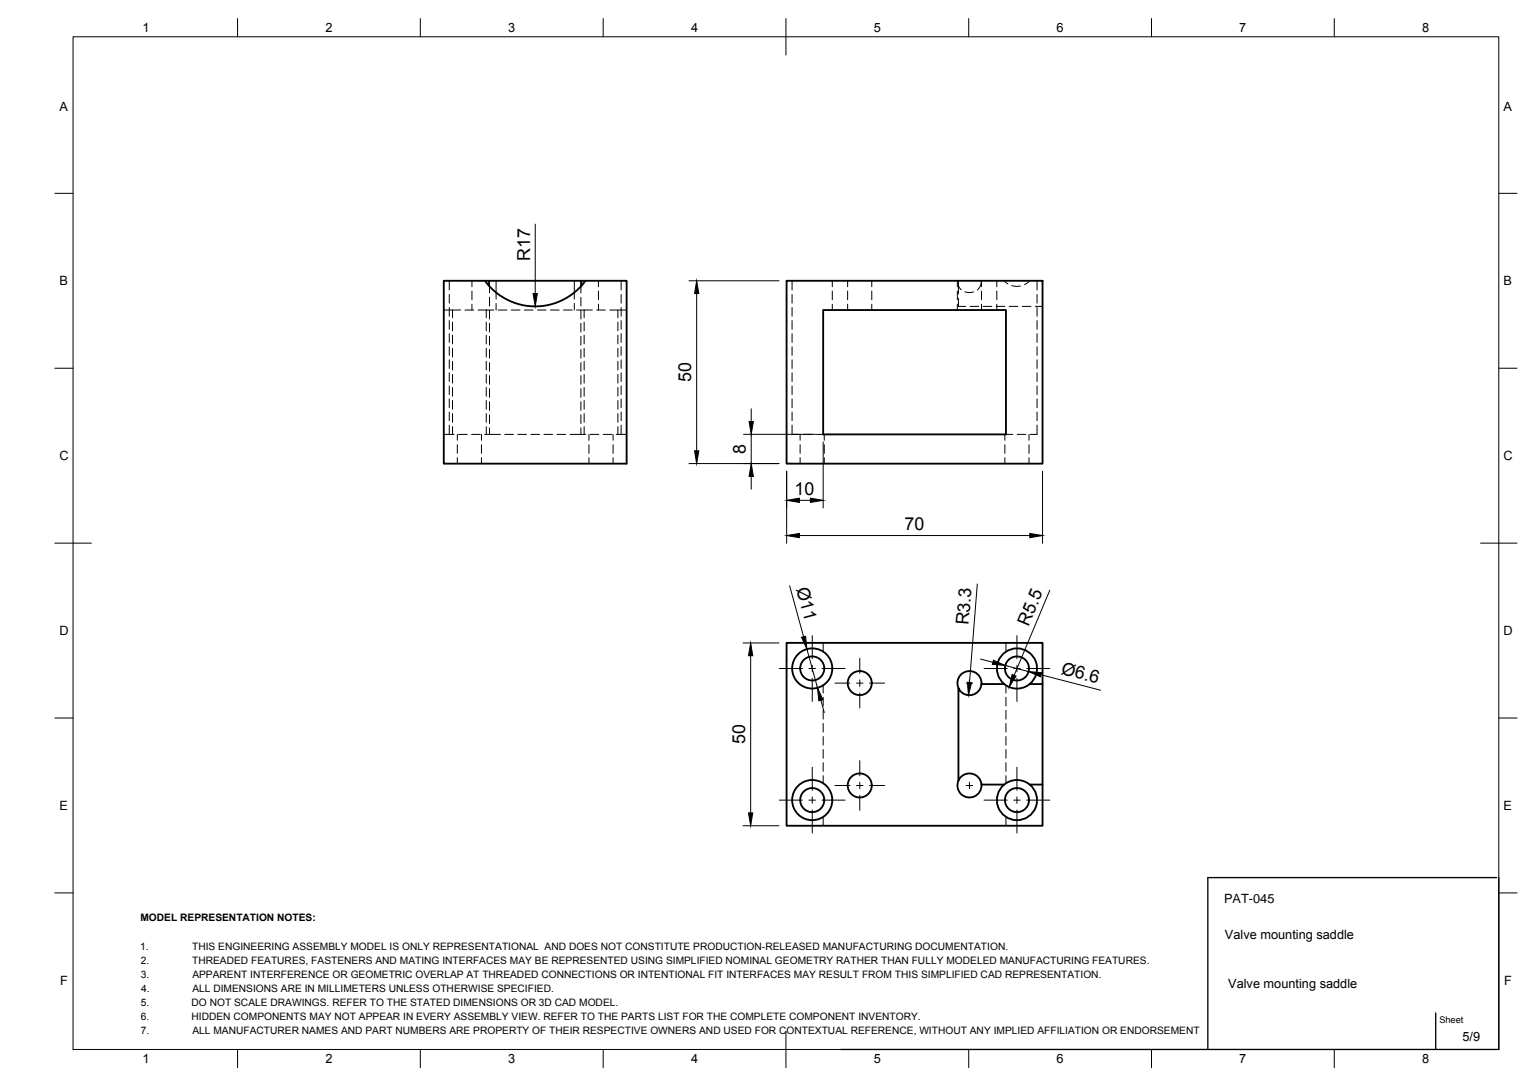
ISO-10303-21;
HEADER;
/* Generated by software containing ST-Developer
 * from STEP Tools, Inc. (www.steptools.com) 
 */

FILE_DESCRIPTION(
/* description */ ('Gauge isolation and snubber set'),
/* implementation_level */ '2;1');

FILE_NAME(
/* name */ 'Valve mounting saddle.step',
/* time_stamp */ '2026-10-29T16:58:15-07:00',
/* author */ (''),
/* organization */ (''),
/* preprocessor_version */ 'ST-DEVELOPER v20.2',
/* originating_system */ 'Autodesk Translation Framework v15.17.0.0',
/* authorisation */ '');

FILE_SCHEMA (('AUTOMOTIVE_DESIGN { 1 0 10303 214 3 1 1 }'));
ENDSEC;

DATA;
#10=MECHANICAL_DESIGN_GEOMETRIC_PRESENTATION_REPRESENTATION('',(#94),#4043);
#78=SHAPE_REPRESENTATION_RELATIONSHIP('SRR','None',#4085,#86);
#86=ADVANCED_BREP_SHAPE_REPRESENTATION('',(#104),#4037);
#94=STYLED_ITEM('',(#4211),#104);
#104=MANIFOLD_SOLID_BREP('Body1',#2211);
#128=FACE_BOUND('',#436,.T.);
#129=FACE_BOUND('',#437,.T.);
#130=FACE_BOUND('',#438,.T.);
#131=FACE_BOUND('',#439,.T.);
#132=FACE_BOUND('',#442,.T.);
#133=FACE_BOUND('',#443,.T.);
#134=FACE_BOUND('',#444,.T.);
#135=FACE_BOUND('',#445,.T.);
#136=FACE_BOUND('',#460,.T.);
#137=FACE_BOUND('',#462,.T.);
#138=FACE_BOUND('',#463,.T.);
#139=FACE_BOUND('',#464,.T.);
#140=FACE_BOUND('',#465,.T.);
#141=FACE_BOUND('',#467,.T.);
#142=FACE_BOUND('',#470,.T.);
#143=FACE_BOUND('',#471,.T.);
#144=FACE_BOUND('',#472,.T.);
#145=FACE_BOUND('',#473,.T.);
#160=B_SPLINE_CURVE_WITH_KNOTS('',3,(#3540,#3541,#3542,#3543,#3544,#3545,
#3546,#3547,#3548,#3549,#3550,#3551,#3552,#3553,#3554,#3555,#3556,#3557,
#3558,#3559),.UNSPECIFIED.,.F.,.F.,(4,2,2,2,2,2,2,2,2,4),(2.69569624904958,
2.75192095998156,2.89158432667083,3.02781992201341,3.15222641361202,3.27663290521063,
3.40103939680924,3.52544588840784,3.66168148375042,3.68881758098469),
 .UNSPECIFIED.);
#161=B_SPLINE_CURVE_WITH_KNOTS('',3,(#3563,#3564,#3565,#3566,#3567,#3568,
#3569,#3570,#3571,#3572,#3573,#3574,#3575,#3576),.UNSPECIFIED.,.F.,.F.,
(4,2,2,2,2,2,4),(2.49458037721665,2.67223802177451,2.78657360475194,2.90090918772936,
3.01524477070679,3.12958035368422,3.30723799824207),.UNSPECIFIED.);
#162=B_SPLINE_CURVE_WITH_KNOTS('',3,(#3584,#3585,#3586,#3587,#3588,#3589,
#3590,#3591,#3592,#3593,#3594,#3595,#3596,#3597,#3598),.UNSPECIFIED.,.F.,
 .F.,(4,2,2,3,2,2,4),(-0.40632881051271,-0.228671165954853,-0.114335582977427,
0.,0.114335582977426,0.228671165954853,0.40632881051271),.UNSPECIFIED.);
#163=B_SPLINE_CURVE_WITH_KNOTS('',3,(#3601,#3602,#3603,#3604,#3605,#3606,
#3607,#3608,#3609,#3610,#3611,#3612,#3613,#3614,#3615,#3616,#3617,#3618,
#3619,#3620,#3621),.UNSPECIFIED.,.F.,.F.,(4,2,2,2,3,2,2,2,2,4),(-0.412184675816244,
-0.385048578539797,-0.248812983197217,-0.124406491598609,0.,0.124406491598609,
0.248812983197217,0.385048578539798,0.524711945229068,0.58093665616105),
 .UNSPECIFIED.);
#193=PLANE('',#2401);
#194=PLANE('',#2424);
#195=PLANE('',#2425);
#196=PLANE('',#2435);
#197=PLANE('',#2443);
#198=PLANE('',#2446);
#199=PLANE('',#2447);
#200=PLANE('',#2450);
#201=PLANE('',#2456);
#202=PLANE('',#2461);
#203=PLANE('',#2462);
#204=PLANE('',#2463);
#205=PLANE('',#2464);
#206=PLANE('',#2465);
#207=PLANE('',#2466);
#288=FACE_OUTER_BOUND('',#428,.T.);
#289=FACE_OUTER_BOUND('',#429,.T.);
#290=FACE_OUTER_BOUND('',#430,.T.);
#291=FACE_OUTER_BOUND('',#431,.T.);
#292=FACE_OUTER_BOUND('',#432,.T.);
#293=FACE_OUTER_BOUND('',#433,.T.);
#294=FACE_OUTER_BOUND('',#434,.T.);
#295=FACE_OUTER_BOUND('',#435,.T.);
#296=FACE_OUTER_BOUND('',#440,.T.);
#297=FACE_OUTER_BOUND('',#441,.T.);
#298=FACE_OUTER_BOUND('',#446,.T.);
#299=FACE_OUTER_BOUND('',#447,.T.);
#300=FACE_OUTER_BOUND('',#448,.T.);
#301=FACE_OUTER_BOUND('',#449,.T.);
#302=FACE_OUTER_BOUND('',#450,.T.);
#303=FACE_OUTER_BOUND('',#451,.T.);
#304=FACE_OUTER_BOUND('',#452,.T.);
#305=FACE_OUTER_BOUND('',#453,.T.);
#306=FACE_OUTER_BOUND('',#454,.T.);
#307=FACE_OUTER_BOUND('',#455,.T.);
#308=FACE_OUTER_BOUND('',#456,.T.);
#309=FACE_OUTER_BOUND('',#457,.T.);
#310=FACE_OUTER_BOUND('',#458,.T.);
#311=FACE_OUTER_BOUND('',#459,.T.);
#312=FACE_OUTER_BOUND('',#461,.T.);
#313=FACE_OUTER_BOUND('',#466,.T.);
#314=FACE_OUTER_BOUND('',#468,.T.);
#315=FACE_OUTER_BOUND('',#469,.T.);
#428=EDGE_LOOP('',(#1659,#1660,#1661,#1662));
#429=EDGE_LOOP('',(#1663,#1664,#1665,#1666,#1667,#1668,#1669,#1670,#1671,
#1672));
#430=EDGE_LOOP('',(#1673,#1674,#1675,#1676,#1677,#1678,#1679,#1680,#1681,
#1682));
#431=EDGE_LOOP('',(#1683,#1684,#1685,#1686,#1687,#1688,#1689));
#432=EDGE_LOOP('',(#1690,#1691,#1692,#1693,#1694,#1695,#1696));
#433=EDGE_LOOP('',(#1697,#1698,#1699,#1700,#1701,#1702,#1703,#1704));
#434=EDGE_LOOP('',(#1705,#1706,#1707,#1708));
#435=EDGE_LOOP('',(#1709,#1710,#1711,#1712,#1713,#1714,#1715,#1716,#1717,
#1718,#1719,#1720,#1721,#1722));
#436=EDGE_LOOP('',(#1723));
#437=EDGE_LOOP('',(#1724));
#438=EDGE_LOOP('',(#1725));
#439=EDGE_LOOP('',(#1726));
#440=EDGE_LOOP('',(#1727,#1728,#1729,#1730));
#441=EDGE_LOOP('',(#1731,#1732,#1733,#1734,#1735,#1736,#1737,#1738,#1739,
#1740,#1741,#1742,#1743,#1744));
#442=EDGE_LOOP('',(#1745));
#443=EDGE_LOOP('',(#1746));
#444=EDGE_LOOP('',(#1747));
#445=EDGE_LOOP('',(#1748));
#446=EDGE_LOOP('',(#1749,#1750,#1751,#1752,#1753,#1754,#1755,#1756));
#447=EDGE_LOOP('',(#1757,#1758,#1759,#1760));
#448=EDGE_LOOP('',(#1761,#1762,#1763,#1764));
#449=EDGE_LOOP('',(#1765,#1766,#1767,#1768));
#450=EDGE_LOOP('',(#1769,#1770,#1771,#1772));
#451=EDGE_LOOP('',(#1773,#1774,#1775,#1776));
#452=EDGE_LOOP('',(#1777,#1778,#1779,#1780));
#453=EDGE_LOOP('',(#1781,#1782,#1783,#1784,#1785,#1786,#1787,#1788,#1789,
#1790));
#454=EDGE_LOOP('',(#1791,#1792,#1793,#1794));
#455=EDGE_LOOP('',(#1795,#1796,#1797,#1798));
#456=EDGE_LOOP('',(#1799,#1800,#1801,#1802));
#457=EDGE_LOOP('',(#1803,#1804,#1805,#1806));
#458=EDGE_LOOP('',(#1807,#1808,#1809,#1810));
#459=EDGE_LOOP('',(#1811,#1812,#1813,#1814));
#460=EDGE_LOOP('',(#1815,#1816,#1817,#1818));
#461=EDGE_LOOP('',(#1819,#1820,#1821,#1822,#1823,#1824,#1825,#1826,#1827,
#1828,#1829,#1830,#1831,#1832,#1833,#1834,#1835,#1836));
#462=EDGE_LOOP('',(#1837));
#463=EDGE_LOOP('',(#1838));
#464=EDGE_LOOP('',(#1839));
#465=EDGE_LOOP('',(#1840));
#466=EDGE_LOOP('',(#1841,#1842,#1843,#1844));
#467=EDGE_LOOP('',(#1845,#1846,#1847,#1848));
#468=EDGE_LOOP('',(#1849,#1850,#1851,#1852,#1853,#1854));
#469=EDGE_LOOP('',(#1855,#1856,#1857,#1858));
#470=EDGE_LOOP('',(#1859));
#471=EDGE_LOOP('',(#1860));
#472=EDGE_LOOP('',(#1861));
#473=EDGE_LOOP('',(#1862));
#571=CIRCLE('',#2402,1.7);
#572=CIRCLE('',#2404,1.7);
#573=CIRCLE('',#2406,0.55);
#574=CIRCLE('',#2407,0.55);
#575=CIRCLE('',#2408,0.55);
#576=CIRCLE('',#2409,0.55);
#577=CIRCLE('',#2410,0.55);
#578=CIRCLE('',#2412,0.33);
#579=CIRCLE('',#2413,0.33);
#580=CIRCLE('',#2414,0.33);
#581=CIRCLE('',#2416,0.33);
#582=CIRCLE('',#2417,0.33);
#583=CIRCLE('',#2418,0.33);
#584=CIRCLE('',#2420,0.55);
#585=CIRCLE('',#2421,0.55);
#586=CIRCLE('',#2422,0.55);
#587=CIRCLE('',#2423,0.55);
#588=CIRCLE('',#2426,0.55);
#589=CIRCLE('',#2427,0.55);
#590=CIRCLE('',#2428,0.55);
#591=CIRCLE('',#2429,0.33);
#592=CIRCLE('',#2430,0.33);
#593=CIRCLE('',#2431,0.33);
#594=CIRCLE('',#2432,0.33);
#595=CIRCLE('',#2434,0.33);
#596=CIRCLE('',#2436,0.55);
#597=CIRCLE('',#2437,0.55);
#598=CIRCLE('',#2438,0.55);
#599=CIRCLE('',#2439,0.33);
#600=CIRCLE('',#2440,0.33);
#601=CIRCLE('',#2442,0.55);
#602=CIRCLE('',#2445,0.33);
#603=CIRCLE('',#2449,0.33);
#604=CIRCLE('',#2452,0.55);
#605=CIRCLE('',#2453,0.55);
#606=CIRCLE('',#2455,0.33);
#607=CIRCLE('',#2458,0.33);
#608=CIRCLE('',#2460,0.33);
#685=LINE('',#3532,#856);
#686=LINE('',#3536,#857);
#687=LINE('',#3537,#858);
#688=LINE('',#3561,#859);
#689=LINE('',#3578,#860);
#690=LINE('',#3582,#861);
#691=LINE('',#3600,#862);
#692=LINE('',#3625,#863);
#693=LINE('',#3629,#864);
#694=LINE('',#3633,#865);
#695=LINE('',#3641,#866);
#696=LINE('',#3648,#867);
#697=LINE('',#3654,#868);
#698=LINE('',#3658,#869);
#699=LINE('',#3663,#870);
#700=LINE('',#3667,#871);
#701=LINE('',#3669,#872);
#702=LINE('',#3670,#873);
#703=LINE('',#3673,#874);
#704=LINE('',#3675,#875);
#705=LINE('',#3676,#876);
#706=LINE('',#3678,#877);
#707=LINE('',#3684,#878);
#708=LINE('',#3686,#879);
#709=LINE('',#3688,#880);
#710=LINE('',#3701,#881);
#711=LINE('',#3708,#882);
#712=LINE('',#3710,#883);
#713=LINE('',#3712,#884);
#714=LINE('',#3715,#885);
#715=LINE('',#3717,#886);
#716=LINE('',#3719,#887);
#717=LINE('',#3720,#888);
#718=LINE('',#3726,#889);
#719=LINE('',#3728,#890);
#720=LINE('',#3731,#891);
#721=LINE('',#3735,#892);
#722=LINE('',#3737,#893);
#723=LINE('',#3739,#894);
#724=LINE('',#3743,#895);
#725=LINE('',#3745,#896);
#726=LINE('',#3747,#897);
#727=LINE('',#3749,#898);
#728=LINE('',#3755,#899);
#729=LINE('',#3757,#900);
#730=LINE('',#3760,#901);
#731=LINE('',#3764,#902);
#732=LINE('',#3769,#903);
#733=LINE('',#3771,#904);
#734=LINE('',#3773,#905);
#735=LINE('',#3774,#906);
#736=LINE('',#3777,#907);
#737=LINE('',#3779,#908);
#738=LINE('',#3780,#909);
#739=LINE('',#3782,#910);
#740=LINE('',#3784,#911);
#741=LINE('',#3785,#912);
#742=LINE('',#3788,#913);
#743=LINE('',#3789,#914);
#744=LINE('',#3791,#915);
#856=VECTOR('',#2798,1.);
#857=VECTOR('',#2801,1.);
#858=VECTOR('',#2802,1.);
#859=VECTOR('',#2805,1.);
#860=VECTOR('',#2806,1.);
#861=VECTOR('',#2809,1.);
#862=VECTOR('',#2810,1.);
#863=VECTOR('',#2813,1.);
#864=VECTOR('',#2816,1.);
#865=VECTOR('',#2819,0.55);
#866=VECTOR('',#2830,0.33);
#867=VECTOR('',#2839,0.33);
#868=VECTOR('',#2846,1.);
#869=VECTOR('',#2849,0.55);
#870=VECTOR('',#2854,1.);
#871=VECTOR('',#2859,1.);
#872=VECTOR('',#2860,1.);
#873=VECTOR('',#2861,1.);
#874=VECTOR('',#2864,1.);
#875=VECTOR('',#2865,1.);
#876=VECTOR('',#2866,1.);
#877=VECTOR('',#2867,1.);
#878=VECTOR('',#2872,1.);
#879=VECTOR('',#2873,1.);
#880=VECTOR('',#2874,1.);
#881=VECTOR('',#2889,0.33);
#882=VECTOR('',#2896,1.);
#883=VECTOR('',#2897,1.);
#884=VECTOR('',#2898,1.);
#885=VECTOR('',#2901,1.);
#886=VECTOR('',#2902,1.);
#887=VECTOR('',#2903,1.);
#888=VECTOR('',#2904,1.);
#889=VECTOR('',#2911,1.);
#890=VECTOR('',#2912,0.55);
#891=VECTOR('',#2917,1.);
#892=VECTOR('',#2922,0.33);
#893=VECTOR('',#2925,1.);
#894=VECTOR('',#2928,1.);
#895=VECTOR('',#2933,0.33);
#896=VECTOR('',#2936,1.);
#897=VECTOR('',#2939,1.);
#898=VECTOR('',#2940,0.55);
#899=VECTOR('',#2949,0.33);
#900=VECTOR('',#2952,1.);
#901=VECTOR('',#2955,0.33);
#902=VECTOR('',#2960,0.33);
#903=VECTOR('',#2965,1.);
#904=VECTOR('',#2966,1.);
#905=VECTOR('',#2967,1.);
#906=VECTOR('',#2968,1.);
#907=VECTOR('',#2971,1.);
#908=VECTOR('',#2972,1.);
#909=VECTOR('',#2973,1.);
#910=VECTOR('',#2976,1.);
#911=VECTOR('',#2977,1.);
#912=VECTOR('',#2978,1.);
#913=VECTOR('',#2981,1.);
#914=VECTOR('',#2982,1.);
#915=VECTOR('',#2985,1.);
#1042=VERTEX_POINT('',#3530);
#1043=VERTEX_POINT('',#3531);
#1044=VERTEX_POINT('',#3533);
#1045=VERTEX_POINT('',#3535);
#1046=VERTEX_POINT('',#3539);
#1047=VERTEX_POINT('',#3560);
#1048=VERTEX_POINT('',#3562);
#1049=VERTEX_POINT('',#3577);
#1050=VERTEX_POINT('',#3579);
#1051=VERTEX_POINT('',#3581);
#1052=VERTEX_POINT('',#3583);
#1053=VERTEX_POINT('',#3599);
#1054=VERTEX_POINT('',#3623);
#1055=VERTEX_POINT('',#3624);
#1056=VERTEX_POINT('',#3626);
#1057=VERTEX_POINT('',#3628);
#1058=VERTEX_POINT('',#3630);
#1059=VERTEX_POINT('',#3632);
#1060=VERTEX_POINT('',#3638);
#1061=VERTEX_POINT('',#3640);
#1062=VERTEX_POINT('',#3645);
#1063=VERTEX_POINT('',#3647);
#1064=VERTEX_POINT('',#3652);
#1065=VERTEX_POINT('',#3653);
#1066=VERTEX_POINT('',#3655);
#1067=VERTEX_POINT('',#3657);
#1068=VERTEX_POINT('',#3660);
#1069=VERTEX_POINT('',#3662);
#1070=VERTEX_POINT('',#3666);
#1071=VERTEX_POINT('',#3668);
#1072=VERTEX_POINT('',#3672);
#1073=VERTEX_POINT('',#3674);
#1074=VERTEX_POINT('',#3677);
#1075=VERTEX_POINT('',#3679);
#1076=VERTEX_POINT('',#3681);
#1077=VERTEX_POINT('',#3683);
#1078=VERTEX_POINT('',#3685);
#1079=VERTEX_POINT('',#3687);
#1080=VERTEX_POINT('',#3690);
#1081=VERTEX_POINT('',#3692);
#1082=VERTEX_POINT('',#3694);
#1083=VERTEX_POINT('',#3696);
#1084=VERTEX_POINT('',#3699);
#1085=VERTEX_POINT('',#3703);
#1086=VERTEX_POINT('',#3705);
#1087=VERTEX_POINT('',#3707);
#1088=VERTEX_POINT('',#3709);
#1089=VERTEX_POINT('',#3711);
#1090=VERTEX_POINT('',#3713);
#1091=VERTEX_POINT('',#3716);
#1092=VERTEX_POINT('',#3718);
#1093=VERTEX_POINT('',#3721);
#1094=VERTEX_POINT('',#3723);
#1095=VERTEX_POINT('',#3727);
#1096=VERTEX_POINT('',#3733);
#1097=VERTEX_POINT('',#3741);
#1098=VERTEX_POINT('',#3748);
#1099=VERTEX_POINT('',#3753);
#1100=VERTEX_POINT('',#3759);
#1101=VERTEX_POINT('',#3763);
#1102=VERTEX_POINT('',#3767);
#1103=VERTEX_POINT('',#3768);
#1104=VERTEX_POINT('',#3770);
#1105=VERTEX_POINT('',#3772);
#1106=VERTEX_POINT('',#3776);
#1107=VERTEX_POINT('',#3778);
#1108=VERTEX_POINT('',#3783);
#1109=VERTEX_POINT('',#3787);
#1268=EDGE_CURVE('',#1042,#1043,#685,.T.);
#1269=EDGE_CURVE('',#1044,#1042,#571,.T.);
#1270=EDGE_CURVE('',#1045,#1044,#686,.T.);
#1271=EDGE_CURVE('',#1043,#1045,#687,.T.);
#1272=EDGE_CURVE('',#1046,#1042,#160,.T.);
#1273=EDGE_CURVE('',#1047,#1046,#688,.T.);
#1274=EDGE_CURVE('',#1048,#1047,#161,.T.);
#1275=EDGE_CURVE('',#1049,#1048,#689,.T.);
#1276=EDGE_CURVE('',#1050,#1049,#572,.T.);
#1277=EDGE_CURVE('',#1051,#1050,#690,.T.);
#1278=EDGE_CURVE('',#1052,#1051,#162,.T.);
#1279=EDGE_CURVE('',#1053,#1052,#691,.T.);
#1280=EDGE_CURVE('',#1044,#1053,#163,.T.);
#1281=EDGE_CURVE('',#1054,#1055,#692,.T.);
#1282=EDGE_CURVE('',#1056,#1054,#573,.T.);
#1283=EDGE_CURVE('',#1057,#1056,#693,.T.);
#1284=EDGE_CURVE('',#1058,#1057,#574,.T.);
#1285=EDGE_CURVE('',#1058,#1059,#694,.T.);
#1286=EDGE_CURVE('',#1048,#1059,#575,.T.);
#1287=EDGE_CURVE('',#1059,#1047,#576,.T.);
#1288=EDGE_CURVE('',#1055,#1058,#577,.T.);
#1289=EDGE_CURVE('',#1060,#1060,#578,.T.);
#1290=EDGE_CURVE('',#1060,#1061,#695,.T.);
#1291=EDGE_CURVE('',#1046,#1061,#579,.T.);
#1292=EDGE_CURVE('',#1061,#1043,#580,.T.);
#1293=EDGE_CURVE('',#1062,#1062,#581,.T.);
#1294=EDGE_CURVE('',#1062,#1063,#696,.T.);
#1295=EDGE_CURVE('',#1045,#1063,#582,.T.);
#1296=EDGE_CURVE('',#1063,#1053,#583,.T.);
#1297=EDGE_CURVE('',#1064,#1065,#697,.T.);
#1298=EDGE_CURVE('',#1066,#1064,#584,.T.);
#1299=EDGE_CURVE('',#1066,#1067,#698,.T.);
#1300=EDGE_CURVE('',#1067,#1067,#585,.T.);
#1301=EDGE_CURVE('',#1068,#1066,#586,.T.);
#1302=EDGE_CURVE('',#1069,#1068,#699,.T.);
#1303=EDGE_CURVE('',#1065,#1069,#587,.T.);
#1304=EDGE_CURVE('',#1070,#1065,#700,.T.);
#1305=EDGE_CURVE('',#1070,#1071,#701,.T.);
#1306=EDGE_CURVE('',#1071,#1064,#702,.T.);
#1307=EDGE_CURVE('',#1069,#1072,#703,.T.);
#1308=EDGE_CURVE('',#1072,#1073,#704,.T.);
#1309=EDGE_CURVE('',#1073,#1055,#705,.T.);
#1310=EDGE_CURVE('',#1057,#1074,#706,.T.);
#1311=EDGE_CURVE('',#1074,#1075,#588,.T.);
#1312=EDGE_CURVE('',#1075,#1076,#589,.T.);
#1313=EDGE_CURVE('',#1076,#1077,#707,.T.);
#1314=EDGE_CURVE('',#1077,#1078,#708,.T.);
#1315=EDGE_CURVE('',#1078,#1079,#709,.T.);
#1316=EDGE_CURVE('',#1079,#1070,#590,.T.);
#1317=EDGE_CURVE('',#1080,#1080,#591,.T.);
#1318=EDGE_CURVE('',#1081,#1081,#592,.T.);
#1319=EDGE_CURVE('',#1082,#1082,#593,.T.);
#1320=EDGE_CURVE('',#1083,#1083,#594,.T.);
#1321=EDGE_CURVE('',#1084,#1084,#595,.T.);
#1322=EDGE_CURVE('',#1084,#1083,#710,.T.);
#1323=EDGE_CURVE('',#1071,#1085,#596,.T.);
#1324=EDGE_CURVE('',#1085,#1086,#597,.T.);
#1325=EDGE_CURVE('',#1087,#1086,#711,.T.);
#1326=EDGE_CURVE('',#1088,#1087,#712,.T.);
#1327=EDGE_CURVE('',#1089,#1088,#713,.T.);
#1328=EDGE_CURVE('',#1089,#1090,#598,.T.);
#1329=EDGE_CURVE('',#1056,#1090,#714,.T.);
#1330=EDGE_CURVE('',#1091,#1054,#715,.T.);
#1331=EDGE_CURVE('',#1092,#1091,#716,.T.);
#1332=EDGE_CURVE('',#1068,#1092,#717,.T.);
#1333=EDGE_CURVE('',#1093,#1093,#599,.T.);
#1334=EDGE_CURVE('',#1094,#1094,#600,.T.);
#1335=EDGE_CURVE('',#1086,#1079,#718,.T.);
#1336=EDGE_CURVE('',#1085,#1095,#719,.T.);
#1337=EDGE_CURVE('',#1095,#1095,#601,.T.);
#1338=EDGE_CURVE('',#1087,#1078,#720,.T.);
#1339=EDGE_CURVE('',#1096,#1096,#602,.T.);
#1340=EDGE_CURVE('',#1096,#1080,#721,.T.);
#1341=EDGE_CURVE('',#1072,#1092,#722,.T.);
#1342=EDGE_CURVE('',#1073,#1091,#723,.T.);
#1343=EDGE_CURVE('',#1097,#1097,#603,.T.);
#1344=EDGE_CURVE('',#1097,#1082,#724,.T.);
#1345=EDGE_CURVE('',#1090,#1074,#725,.T.);
#1346=EDGE_CURVE('',#1076,#1089,#726,.T.);
#1347=EDGE_CURVE('',#1075,#1098,#727,.T.);
#1348=EDGE_CURVE('',#1052,#1098,#604,.T.);
#1349=EDGE_CURVE('',#1098,#1051,#605,.T.);
#1350=EDGE_CURVE('',#1099,#1099,#606,.T.);
#1351=EDGE_CURVE('',#1099,#1081,#728,.T.);
#1352=EDGE_CURVE('',#1088,#1077,#729,.T.);
#1353=EDGE_CURVE('',#1094,#1100,#730,.T.);
#1354=EDGE_CURVE('',#1100,#1100,#607,.T.);
#1355=EDGE_CURVE('',#1093,#1101,#731,.T.);
#1356=EDGE_CURVE('',#1101,#1101,#608,.T.);
#1357=EDGE_CURVE('',#1102,#1103,#732,.T.);
#1358=EDGE_CURVE('',#1102,#1104,#733,.T.);
#1359=EDGE_CURVE('',#1104,#1105,#734,.T.);
#1360=EDGE_CURVE('',#1105,#1103,#735,.T.);
#1361=EDGE_CURVE('',#1106,#1103,#736,.T.);
#1362=EDGE_CURVE('',#1107,#1106,#737,.T.);
#1363=EDGE_CURVE('',#1107,#1102,#738,.T.);
#1364=EDGE_CURVE('',#1050,#1106,#739,.T.);
#1365=EDGE_CURVE('',#1108,#1105,#740,.T.);
#1366=EDGE_CURVE('',#1108,#1049,#741,.T.);
#1367=EDGE_CURVE('',#1104,#1109,#742,.T.);
#1368=EDGE_CURVE('',#1109,#1108,#743,.T.);
#1369=EDGE_CURVE('',#1109,#1107,#744,.T.);
#1659=ORIENTED_EDGE('',*,*,#1268,.F.);
#1660=ORIENTED_EDGE('',*,*,#1269,.F.);
#1661=ORIENTED_EDGE('',*,*,#1270,.F.);
#1662=ORIENTED_EDGE('',*,*,#1271,.F.);
#1663=ORIENTED_EDGE('',*,*,#1272,.F.);
#1664=ORIENTED_EDGE('',*,*,#1273,.F.);
#1665=ORIENTED_EDGE('',*,*,#1274,.F.);
#1666=ORIENTED_EDGE('',*,*,#1275,.F.);
#1667=ORIENTED_EDGE('',*,*,#1276,.F.);
#1668=ORIENTED_EDGE('',*,*,#1277,.F.);
#1669=ORIENTED_EDGE('',*,*,#1278,.F.);
#1670=ORIENTED_EDGE('',*,*,#1279,.F.);
#1671=ORIENTED_EDGE('',*,*,#1280,.F.);
#1672=ORIENTED_EDGE('',*,*,#1269,.T.);
#1673=ORIENTED_EDGE('',*,*,#1281,.F.);
#1674=ORIENTED_EDGE('',*,*,#1282,.F.);
#1675=ORIENTED_EDGE('',*,*,#1283,.F.);
#1676=ORIENTED_EDGE('',*,*,#1284,.F.);
#1677=ORIENTED_EDGE('',*,*,#1285,.T.);
#1678=ORIENTED_EDGE('',*,*,#1286,.F.);
#1679=ORIENTED_EDGE('',*,*,#1274,.T.);
#1680=ORIENTED_EDGE('',*,*,#1287,.F.);
#1681=ORIENTED_EDGE('',*,*,#1285,.F.);
#1682=ORIENTED_EDGE('',*,*,#1288,.F.);
#1683=ORIENTED_EDGE('',*,*,#1289,.F.);
#1684=ORIENTED_EDGE('',*,*,#1290,.T.);
#1685=ORIENTED_EDGE('',*,*,#1291,.F.);
#1686=ORIENTED_EDGE('',*,*,#1272,.T.);
#1687=ORIENTED_EDGE('',*,*,#1268,.T.);
#1688=ORIENTED_EDGE('',*,*,#1292,.F.);
#1689=ORIENTED_EDGE('',*,*,#1290,.F.);
#1690=ORIENTED_EDGE('',*,*,#1293,.F.);
#1691=ORIENTED_EDGE('',*,*,#1294,.T.);
#1692=ORIENTED_EDGE('',*,*,#1295,.F.);
#1693=ORIENTED_EDGE('',*,*,#1270,.T.);
#1694=ORIENTED_EDGE('',*,*,#1280,.T.);
#1695=ORIENTED_EDGE('',*,*,#1296,.F.);
#1696=ORIENTED_EDGE('',*,*,#1294,.F.);
#1697=ORIENTED_EDGE('',*,*,#1297,.F.);
#1698=ORIENTED_EDGE('',*,*,#1298,.F.);
#1699=ORIENTED_EDGE('',*,*,#1299,.T.);
#1700=ORIENTED_EDGE('',*,*,#1300,.F.);
#1701=ORIENTED_EDGE('',*,*,#1299,.F.);
#1702=ORIENTED_EDGE('',*,*,#1301,.F.);
#1703=ORIENTED_EDGE('',*,*,#1302,.F.);
#1704=ORIENTED_EDGE('',*,*,#1303,.F.);
#1705=ORIENTED_EDGE('',*,*,#1297,.T.);
#1706=ORIENTED_EDGE('',*,*,#1304,.F.);
#1707=ORIENTED_EDGE('',*,*,#1305,.T.);
#1708=ORIENTED_EDGE('',*,*,#1306,.T.);
#1709=ORIENTED_EDGE('',*,*,#1307,.T.);
#1710=ORIENTED_EDGE('',*,*,#1308,.T.);
#1711=ORIENTED_EDGE('',*,*,#1309,.T.);
#1712=ORIENTED_EDGE('',*,*,#1288,.T.);
#1713=ORIENTED_EDGE('',*,*,#1284,.T.);
#1714=ORIENTED_EDGE('',*,*,#1310,.T.);
#1715=ORIENTED_EDGE('',*,*,#1311,.T.);
#1716=ORIENTED_EDGE('',*,*,#1312,.T.);
#1717=ORIENTED_EDGE('',*,*,#1313,.T.);
#1718=ORIENTED_EDGE('',*,*,#1314,.T.);
#1719=ORIENTED_EDGE('',*,*,#1315,.T.);
#1720=ORIENTED_EDGE('',*,*,#1316,.T.);
#1721=ORIENTED_EDGE('',*,*,#1304,.T.);
#1722=ORIENTED_EDGE('',*,*,#1303,.T.);
#1723=ORIENTED_EDGE('',*,*,#1317,.F.);
#1724=ORIENTED_EDGE('',*,*,#1318,.F.);
#1725=ORIENTED_EDGE('',*,*,#1319,.T.);
#1726=ORIENTED_EDGE('',*,*,#1320,.T.);
#1727=ORIENTED_EDGE('',*,*,#1321,.F.);
#1728=ORIENTED_EDGE('',*,*,#1322,.T.);
#1729=ORIENTED_EDGE('',*,*,#1320,.F.);
#1730=ORIENTED_EDGE('',*,*,#1322,.F.);
#1731=ORIENTED_EDGE('',*,*,#1301,.T.);
#1732=ORIENTED_EDGE('',*,*,#1298,.T.);
#1733=ORIENTED_EDGE('',*,*,#1306,.F.);
#1734=ORIENTED_EDGE('',*,*,#1323,.T.);
#1735=ORIENTED_EDGE('',*,*,#1324,.T.);
#1736=ORIENTED_EDGE('',*,*,#1325,.F.);
#1737=ORIENTED_EDGE('',*,*,#1326,.F.);
#1738=ORIENTED_EDGE('',*,*,#1327,.F.);
#1739=ORIENTED_EDGE('',*,*,#1328,.T.);
#1740=ORIENTED_EDGE('',*,*,#1329,.F.);
#1741=ORIENTED_EDGE('',*,*,#1282,.T.);
#1742=ORIENTED_EDGE('',*,*,#1330,.F.);
#1743=ORIENTED_EDGE('',*,*,#1331,.F.);
#1744=ORIENTED_EDGE('',*,*,#1332,.F.);
#1745=ORIENTED_EDGE('',*,*,#1293,.T.);
#1746=ORIENTED_EDGE('',*,*,#1289,.T.);
#1747=ORIENTED_EDGE('',*,*,#1333,.T.);
#1748=ORIENTED_EDGE('',*,*,#1334,.T.);
#1749=ORIENTED_EDGE('',*,*,#1335,.F.);
#1750=ORIENTED_EDGE('',*,*,#1324,.F.);
#1751=ORIENTED_EDGE('',*,*,#1336,.T.);
#1752=ORIENTED_EDGE('',*,*,#1337,.F.);
#1753=ORIENTED_EDGE('',*,*,#1336,.F.);
#1754=ORIENTED_EDGE('',*,*,#1323,.F.);
#1755=ORIENTED_EDGE('',*,*,#1305,.F.);
#1756=ORIENTED_EDGE('',*,*,#1316,.F.);
#1757=ORIENTED_EDGE('',*,*,#1335,.T.);
#1758=ORIENTED_EDGE('',*,*,#1315,.F.);
#1759=ORIENTED_EDGE('',*,*,#1338,.F.);
#1760=ORIENTED_EDGE('',*,*,#1325,.T.);
#1761=ORIENTED_EDGE('',*,*,#1339,.F.);
#1762=ORIENTED_EDGE('',*,*,#1340,.T.);
#1763=ORIENTED_EDGE('',*,*,#1317,.T.);
#1764=ORIENTED_EDGE('',*,*,#1340,.F.);
#1765=ORIENTED_EDGE('',*,*,#1302,.T.);
#1766=ORIENTED_EDGE('',*,*,#1332,.T.);
#1767=ORIENTED_EDGE('',*,*,#1341,.F.);
#1768=ORIENTED_EDGE('',*,*,#1307,.F.);
#1769=ORIENTED_EDGE('',*,*,#1281,.T.);
#1770=ORIENTED_EDGE('',*,*,#1309,.F.);
#1771=ORIENTED_EDGE('',*,*,#1342,.T.);
#1772=ORIENTED_EDGE('',*,*,#1330,.T.);
#1773=ORIENTED_EDGE('',*,*,#1343,.F.);
#1774=ORIENTED_EDGE('',*,*,#1344,.T.);
#1775=ORIENTED_EDGE('',*,*,#1319,.F.);
#1776=ORIENTED_EDGE('',*,*,#1344,.F.);
#1777=ORIENTED_EDGE('',*,*,#1283,.T.);
#1778=ORIENTED_EDGE('',*,*,#1329,.T.);
#1779=ORIENTED_EDGE('',*,*,#1345,.T.);
#1780=ORIENTED_EDGE('',*,*,#1310,.F.);
#1781=ORIENTED_EDGE('',*,*,#1345,.F.);
#1782=ORIENTED_EDGE('',*,*,#1328,.F.);
#1783=ORIENTED_EDGE('',*,*,#1346,.F.);
#1784=ORIENTED_EDGE('',*,*,#1312,.F.);
#1785=ORIENTED_EDGE('',*,*,#1347,.T.);
#1786=ORIENTED_EDGE('',*,*,#1348,.F.);
#1787=ORIENTED_EDGE('',*,*,#1278,.T.);
#1788=ORIENTED_EDGE('',*,*,#1349,.F.);
#1789=ORIENTED_EDGE('',*,*,#1347,.F.);
#1790=ORIENTED_EDGE('',*,*,#1311,.F.);
#1791=ORIENTED_EDGE('',*,*,#1350,.F.);
#1792=ORIENTED_EDGE('',*,*,#1351,.T.);
#1793=ORIENTED_EDGE('',*,*,#1318,.T.);
#1794=ORIENTED_EDGE('',*,*,#1351,.F.);
#1795=ORIENTED_EDGE('',*,*,#1346,.T.);
#1796=ORIENTED_EDGE('',*,*,#1327,.T.);
#1797=ORIENTED_EDGE('',*,*,#1352,.T.);
#1798=ORIENTED_EDGE('',*,*,#1313,.F.);
#1799=ORIENTED_EDGE('',*,*,#1334,.F.);
#1800=ORIENTED_EDGE('',*,*,#1353,.T.);
#1801=ORIENTED_EDGE('',*,*,#1354,.F.);
#1802=ORIENTED_EDGE('',*,*,#1353,.F.);
#1803=ORIENTED_EDGE('',*,*,#1333,.F.);
#1804=ORIENTED_EDGE('',*,*,#1355,.T.);
#1805=ORIENTED_EDGE('',*,*,#1356,.F.);
#1806=ORIENTED_EDGE('',*,*,#1355,.F.);
#1807=ORIENTED_EDGE('',*,*,#1357,.F.);
#1808=ORIENTED_EDGE('',*,*,#1358,.T.);
#1809=ORIENTED_EDGE('',*,*,#1359,.T.);
#1810=ORIENTED_EDGE('',*,*,#1360,.T.);
#1811=ORIENTED_EDGE('',*,*,#1361,.F.);
#1812=ORIENTED_EDGE('',*,*,#1362,.F.);
#1813=ORIENTED_EDGE('',*,*,#1363,.T.);
#1814=ORIENTED_EDGE('',*,*,#1357,.T.);
#1815=ORIENTED_EDGE('',*,*,#1338,.T.);
#1816=ORIENTED_EDGE('',*,*,#1314,.F.);
#1817=ORIENTED_EDGE('',*,*,#1352,.F.);
#1818=ORIENTED_EDGE('',*,*,#1326,.T.);
#1819=ORIENTED_EDGE('',*,*,#1275,.T.);
#1820=ORIENTED_EDGE('',*,*,#1286,.T.);
#1821=ORIENTED_EDGE('',*,*,#1287,.T.);
#1822=ORIENTED_EDGE('',*,*,#1273,.T.);
#1823=ORIENTED_EDGE('',*,*,#1291,.T.);
#1824=ORIENTED_EDGE('',*,*,#1292,.T.);
#1825=ORIENTED_EDGE('',*,*,#1271,.T.);
#1826=ORIENTED_EDGE('',*,*,#1295,.T.);
#1827=ORIENTED_EDGE('',*,*,#1296,.T.);
#1828=ORIENTED_EDGE('',*,*,#1279,.T.);
#1829=ORIENTED_EDGE('',*,*,#1348,.T.);
#1830=ORIENTED_EDGE('',*,*,#1349,.T.);
#1831=ORIENTED_EDGE('',*,*,#1277,.T.);
#1832=ORIENTED_EDGE('',*,*,#1364,.T.);
#1833=ORIENTED_EDGE('',*,*,#1361,.T.);
#1834=ORIENTED_EDGE('',*,*,#1360,.F.);
#1835=ORIENTED_EDGE('',*,*,#1365,.F.);
#1836=ORIENTED_EDGE('',*,*,#1366,.T.);
#1837=ORIENTED_EDGE('',*,*,#1356,.T.);
#1838=ORIENTED_EDGE('',*,*,#1354,.T.);
#1839=ORIENTED_EDGE('',*,*,#1337,.T.);
#1840=ORIENTED_EDGE('',*,*,#1300,.T.);
#1841=ORIENTED_EDGE('',*,*,#1365,.T.);
#1842=ORIENTED_EDGE('',*,*,#1359,.F.);
#1843=ORIENTED_EDGE('',*,*,#1367,.T.);
#1844=ORIENTED_EDGE('',*,*,#1368,.T.);
#1845=ORIENTED_EDGE('',*,*,#1331,.T.);
#1846=ORIENTED_EDGE('',*,*,#1342,.F.);
#1847=ORIENTED_EDGE('',*,*,#1308,.F.);
#1848=ORIENTED_EDGE('',*,*,#1341,.T.);
#1849=ORIENTED_EDGE('',*,*,#1276,.T.);
#1850=ORIENTED_EDGE('',*,*,#1366,.F.);
#1851=ORIENTED_EDGE('',*,*,#1368,.F.);
#1852=ORIENTED_EDGE('',*,*,#1369,.T.);
#1853=ORIENTED_EDGE('',*,*,#1362,.T.);
#1854=ORIENTED_EDGE('',*,*,#1364,.F.);
#1855=ORIENTED_EDGE('',*,*,#1369,.F.);
#1856=ORIENTED_EDGE('',*,*,#1367,.F.);
#1857=ORIENTED_EDGE('',*,*,#1358,.F.);
#1858=ORIENTED_EDGE('',*,*,#1363,.F.);
#1859=ORIENTED_EDGE('',*,*,#1321,.T.);
#1860=ORIENTED_EDGE('',*,*,#1339,.T.);
#1861=ORIENTED_EDGE('',*,*,#1343,.T.);
#1862=ORIENTED_EDGE('',*,*,#1350,.T.);
#2063=CYLINDRICAL_SURFACE('',#2403,1.7);
#2064=CYLINDRICAL_SURFACE('',#2405,0.55);
#2065=CYLINDRICAL_SURFACE('',#2411,0.33);
#2066=CYLINDRICAL_SURFACE('',#2415,0.33);
#2067=CYLINDRICAL_SURFACE('',#2419,0.55);
#2068=CYLINDRICAL_SURFACE('',#2433,0.33);
#2069=CYLINDRICAL_SURFACE('',#2441,0.55);
#2070=CYLINDRICAL_SURFACE('',#2444,0.33);
#2071=CYLINDRICAL_SURFACE('',#2448,0.33);
#2072=CYLINDRICAL_SURFACE('',#2451,0.55);
#2073=CYLINDRICAL_SURFACE('',#2454,0.33);
#2074=CYLINDRICAL_SURFACE('',#2457,0.33);
#2075=CYLINDRICAL_SURFACE('',#2459,0.33);
#2132=ADVANCED_FACE('',(#288),#193,.F.);
#2133=ADVANCED_FACE('',(#289),#2063,.F.);
#2134=ADVANCED_FACE('',(#290),#2064,.F.);
#2135=ADVANCED_FACE('',(#291),#2065,.F.);
#2136=ADVANCED_FACE('',(#292),#2066,.F.);
#2137=ADVANCED_FACE('',(#293),#2067,.F.);
#2138=ADVANCED_FACE('',(#294),#194,.F.);
#2139=ADVANCED_FACE('',(#295,#128,#129,#130,#131),#195,.T.);
#2140=ADVANCED_FACE('',(#296),#2068,.F.);
#2141=ADVANCED_FACE('',(#297,#132,#133,#134,#135),#196,.F.);
#2142=ADVANCED_FACE('',(#298),#2069,.F.);
#2143=ADVANCED_FACE('',(#299),#197,.F.);
#2144=ADVANCED_FACE('',(#300),#2070,.F.);
#2145=ADVANCED_FACE('',(#301),#198,.F.);
#2146=ADVANCED_FACE('',(#302),#199,.T.);
#2147=ADVANCED_FACE('',(#303),#2071,.F.);
#2148=ADVANCED_FACE('',(#304),#200,.T.);
#2149=ADVANCED_FACE('',(#305),#2072,.F.);
#2150=ADVANCED_FACE('',(#306),#2073,.F.);
#2151=ADVANCED_FACE('',(#307),#201,.T.);
#2152=ADVANCED_FACE('',(#308),#2074,.F.);
#2153=ADVANCED_FACE('',(#309),#2075,.F.);
#2154=ADVANCED_FACE('',(#310),#202,.T.);
#2155=ADVANCED_FACE('',(#311,#136),#203,.T.);
#2156=ADVANCED_FACE('',(#312,#137,#138,#139,#140),#204,.T.);
#2157=ADVANCED_FACE('',(#313,#141),#205,.T.);
#2158=ADVANCED_FACE('',(#314),#206,.T.);
#2159=ADVANCED_FACE('',(#315,#142,#143,#144,#145),#207,.F.);
#2211=CLOSED_SHELL('',(#2132,#2133,#2134,#2135,#2136,#2137,#2138,#2139,
#2140,#2141,#2142,#2143,#2144,#2145,#2146,#2147,#2148,#2149,#2150,#2151,
#2152,#2153,#2154,#2155,#2156,#2157,#2158,#2159));
#2400=AXIS2_PLACEMENT_3D('',#3528,#2794,#2795);
#2401=AXIS2_PLACEMENT_3D('',#3529,#2796,#2797);
#2402=AXIS2_PLACEMENT_3D('',#3534,#2799,#2800);
#2403=AXIS2_PLACEMENT_3D('',#3538,#2803,#2804);
#2404=AXIS2_PLACEMENT_3D('',#3580,#2807,#2808);
#2405=AXIS2_PLACEMENT_3D('',#3622,#2811,#2812);
#2406=AXIS2_PLACEMENT_3D('',#3627,#2814,#2815);
#2407=AXIS2_PLACEMENT_3D('',#3631,#2817,#2818);
#2408=AXIS2_PLACEMENT_3D('',#3634,#2820,#2821);
#2409=AXIS2_PLACEMENT_3D('',#3635,#2822,#2823);
#2410=AXIS2_PLACEMENT_3D('',#3636,#2824,#2825);
#2411=AXIS2_PLACEMENT_3D('',#3637,#2826,#2827);
#2412=AXIS2_PLACEMENT_3D('',#3639,#2828,#2829);
#2413=AXIS2_PLACEMENT_3D('',#3642,#2831,#2832);
#2414=AXIS2_PLACEMENT_3D('',#3643,#2833,#2834);
#2415=AXIS2_PLACEMENT_3D('',#3644,#2835,#2836);
#2416=AXIS2_PLACEMENT_3D('',#3646,#2837,#2838);
#2417=AXIS2_PLACEMENT_3D('',#3649,#2840,#2841);
#2418=AXIS2_PLACEMENT_3D('',#3650,#2842,#2843);
#2419=AXIS2_PLACEMENT_3D('',#3651,#2844,#2845);
#2420=AXIS2_PLACEMENT_3D('',#3656,#2847,#2848);
#2421=AXIS2_PLACEMENT_3D('',#3659,#2850,#2851);
#2422=AXIS2_PLACEMENT_3D('',#3661,#2852,#2853);
#2423=AXIS2_PLACEMENT_3D('',#3664,#2855,#2856);
#2424=AXIS2_PLACEMENT_3D('',#3665,#2857,#2858);
#2425=AXIS2_PLACEMENT_3D('',#3671,#2862,#2863);
#2426=AXIS2_PLACEMENT_3D('',#3680,#2868,#2869);
#2427=AXIS2_PLACEMENT_3D('',#3682,#2870,#2871);
#2428=AXIS2_PLACEMENT_3D('',#3689,#2875,#2876);
#2429=AXIS2_PLACEMENT_3D('',#3691,#2877,#2878);
#2430=AXIS2_PLACEMENT_3D('',#3693,#2879,#2880);
#2431=AXIS2_PLACEMENT_3D('',#3695,#2881,#2882);
#2432=AXIS2_PLACEMENT_3D('',#3697,#2883,#2884);
#2433=AXIS2_PLACEMENT_3D('',#3698,#2885,#2886);
#2434=AXIS2_PLACEMENT_3D('',#3700,#2887,#2888);
#2435=AXIS2_PLACEMENT_3D('',#3702,#2890,#2891);
#2436=AXIS2_PLACEMENT_3D('',#3704,#2892,#2893);
#2437=AXIS2_PLACEMENT_3D('',#3706,#2894,#2895);
#2438=AXIS2_PLACEMENT_3D('',#3714,#2899,#2900);
#2439=AXIS2_PLACEMENT_3D('',#3722,#2905,#2906);
#2440=AXIS2_PLACEMENT_3D('',#3724,#2907,#2908);
#2441=AXIS2_PLACEMENT_3D('',#3725,#2909,#2910);
#2442=AXIS2_PLACEMENT_3D('',#3729,#2913,#2914);
#2443=AXIS2_PLACEMENT_3D('',#3730,#2915,#2916);
#2444=AXIS2_PLACEMENT_3D('',#3732,#2918,#2919);
#2445=AXIS2_PLACEMENT_3D('',#3734,#2920,#2921);
#2446=AXIS2_PLACEMENT_3D('',#3736,#2923,#2924);
#2447=AXIS2_PLACEMENT_3D('',#3738,#2926,#2927);
#2448=AXIS2_PLACEMENT_3D('',#3740,#2929,#2930);
#2449=AXIS2_PLACEMENT_3D('',#3742,#2931,#2932);
#2450=AXIS2_PLACEMENT_3D('',#3744,#2934,#2935);
#2451=AXIS2_PLACEMENT_3D('',#3746,#2937,#2938);
#2452=AXIS2_PLACEMENT_3D('',#3750,#2941,#2942);
#2453=AXIS2_PLACEMENT_3D('',#3751,#2943,#2944);
#2454=AXIS2_PLACEMENT_3D('',#3752,#2945,#2946);
#2455=AXIS2_PLACEMENT_3D('',#3754,#2947,#2948);
#2456=AXIS2_PLACEMENT_3D('',#3756,#2950,#2951);
#2457=AXIS2_PLACEMENT_3D('',#3758,#2953,#2954);
#2458=AXIS2_PLACEMENT_3D('',#3761,#2956,#2957);
#2459=AXIS2_PLACEMENT_3D('',#3762,#2958,#2959);
#2460=AXIS2_PLACEMENT_3D('',#3765,#2961,#2962);
#2461=AXIS2_PLACEMENT_3D('',#3766,#2963,#2964);
#2462=AXIS2_PLACEMENT_3D('',#3775,#2969,#2970);
#2463=AXIS2_PLACEMENT_3D('',#3781,#2974,#2975);
#2464=AXIS2_PLACEMENT_3D('',#3786,#2979,#2980);
#2465=AXIS2_PLACEMENT_3D('',#3790,#2983,#2984);
#2466=AXIS2_PLACEMENT_3D('',#3792,#2986,#2987);
#2794=DIRECTION('axis',(0.,0.,1.));
#2795=DIRECTION('refdir',(1.,0.,0.));
#2796=DIRECTION('center_axis',(1.,0.,0.));
#2797=DIRECTION('ref_axis',(0.,0.,-1.));
#2798=DIRECTION('',(0.,0.,1.));
#2799=DIRECTION('center_axis',(1.,0.,0.));
#2800=DIRECTION('ref_axis',(0.,0.,-1.));
#2801=DIRECTION('',(0.,0.,-1.));
#2802=DIRECTION('',(0.,-1.,0.));
#2803=DIRECTION('center_axis',(1.,0.,0.));
#2804=DIRECTION('ref_axis',(0.,0.,-1.));
#2805=DIRECTION('',(1.,0.,0.));
#2806=DIRECTION('',(1.,0.,0.));
#2807=DIRECTION('center_axis',(1.,0.,0.));
#2808=DIRECTION('ref_axis',(0.,0.,-1.));
#2809=DIRECTION('',(-1.,0.,0.));
#2810=DIRECTION('',(-1.,0.,0.));
#2811=DIRECTION('center_axis',(0.,0.,1.));
#2812=DIRECTION('ref_axis',(1.,0.,0.));
#2813=DIRECTION('',(0.,0.,-1.));
#2814=DIRECTION('center_axis',(0.,0.,1.));
#2815=DIRECTION('ref_axis',(1.,0.,0.));
#2816=DIRECTION('',(0.,0.,1.));
#2817=DIRECTION('center_axis',(0.,0.,1.));
#2818=DIRECTION('ref_axis',(1.,0.,0.));
#2819=DIRECTION('',(0.,0.,1.));
#2820=DIRECTION('center_axis',(0.,0.,-1.));
#2821=DIRECTION('ref_axis',(1.,0.,0.));
#2822=DIRECTION('center_axis',(0.,0.,-1.));
#2823=DIRECTION('ref_axis',(1.,0.,0.));
#2824=DIRECTION('center_axis',(0.,0.,1.));
#2825=DIRECTION('ref_axis',(1.,0.,0.));
#2826=DIRECTION('center_axis',(0.,0.,1.));
#2827=DIRECTION('ref_axis',(1.,0.,0.));
#2828=DIRECTION('center_axis',(0.,0.,1.));
#2829=DIRECTION('ref_axis',(1.,0.,0.));
#2830=DIRECTION('',(0.,0.,1.));
#2831=DIRECTION('center_axis',(0.,0.,-1.));
#2832=DIRECTION('ref_axis',(1.,0.,0.));
#2833=DIRECTION('center_axis',(0.,0.,-1.));
#2834=DIRECTION('ref_axis',(1.,0.,0.));
#2835=DIRECTION('center_axis',(0.,0.,1.));
#2836=DIRECTION('ref_axis',(1.,0.,0.));
#2837=DIRECTION('center_axis',(0.,0.,1.));
#2838=DIRECTION('ref_axis',(1.,0.,0.));
#2839=DIRECTION('',(0.,0.,1.));
#2840=DIRECTION('center_axis',(0.,0.,-1.));
#2841=DIRECTION('ref_axis',(1.,0.,0.));
#2842=DIRECTION('center_axis',(0.,0.,-1.));
#2843=DIRECTION('ref_axis',(1.,0.,0.));
#2844=DIRECTION('center_axis',(0.,0.,1.));
#2845=DIRECTION('ref_axis',(1.,0.,0.));
#2846=DIRECTION('',(0.,0.,-1.));
#2847=DIRECTION('center_axis',(0.,0.,1.));
#2848=DIRECTION('ref_axis',(1.,0.,0.));
#2849=DIRECTION('',(0.,0.,1.));
#2850=DIRECTION('center_axis',(0.,0.,-1.));
#2851=DIRECTION('ref_axis',(1.,0.,0.));
#2852=DIRECTION('center_axis',(0.,0.,1.));
#2853=DIRECTION('ref_axis',(1.,0.,0.));
#2854=DIRECTION('',(0.,0.,1.));
#2855=DIRECTION('center_axis',(0.,0.,1.));
#2856=DIRECTION('ref_axis',(1.,0.,0.));
#2857=DIRECTION('center_axis',(1.,0.,0.));
#2858=DIRECTION('ref_axis',(0.,0.,-1.));
#2859=DIRECTION('',(0.,1.,0.));
#2860=DIRECTION('',(0.,0.,1.));
#2861=DIRECTION('',(0.,1.,0.));
#2862=DIRECTION('center_axis',(0.,0.,1.));
#2863=DIRECTION('ref_axis',(1.,0.,0.));
#2864=DIRECTION('',(0.,1.,0.));
#2865=DIRECTION('',(-1.,0.,0.));
#2866=DIRECTION('',(0.,-1.,0.));
#2867=DIRECTION('',(0.,-1.,0.));
#2868=DIRECTION('center_axis',(0.,0.,1.));
#2869=DIRECTION('ref_axis',(1.,0.,0.));
#2870=DIRECTION('center_axis',(0.,0.,1.));
#2871=DIRECTION('ref_axis',(1.,0.,0.));
#2872=DIRECTION('',(0.,-1.,0.));
#2873=DIRECTION('',(1.,0.,0.));
#2874=DIRECTION('',(0.,1.,0.));
#2875=DIRECTION('center_axis',(0.,0.,1.));
#2876=DIRECTION('ref_axis',(1.,0.,0.));
#2877=DIRECTION('center_axis',(0.,0.,1.));
#2878=DIRECTION('ref_axis',(1.,0.,0.));
#2879=DIRECTION('center_axis',(0.,0.,1.));
#2880=DIRECTION('ref_axis',(1.,0.,0.));
#2881=DIRECTION('center_axis',(0.,0.,-1.));
#2882=DIRECTION('ref_axis',(1.,0.,0.));
#2883=DIRECTION('center_axis',(0.,0.,-1.));
#2884=DIRECTION('ref_axis',(1.,0.,0.));
#2885=DIRECTION('center_axis',(0.,0.,1.));
#2886=DIRECTION('ref_axis',(1.,0.,0.));
#2887=DIRECTION('center_axis',(0.,0.,1.));
#2888=DIRECTION('ref_axis',(1.,0.,0.));
#2889=DIRECTION('',(0.,0.,1.));
#2890=DIRECTION('center_axis',(0.,0.,1.));
#2891=DIRECTION('ref_axis',(1.,0.,0.));
#2892=DIRECTION('center_axis',(0.,0.,1.));
#2893=DIRECTION('ref_axis',(1.,0.,0.));
#2894=DIRECTION('center_axis',(0.,0.,1.));
#2895=DIRECTION('ref_axis',(1.,0.,0.));
#2896=DIRECTION('',(0.,1.,0.));
#2897=DIRECTION('',(1.,0.,0.));
#2898=DIRECTION('',(0.,-1.,0.));
#2899=DIRECTION('center_axis',(0.,0.,1.));
#2900=DIRECTION('ref_axis',(1.,0.,0.));
#2901=DIRECTION('',(0.,-1.,0.));
#2902=DIRECTION('',(0.,-1.,0.));
#2903=DIRECTION('',(-1.,0.,0.));
#2904=DIRECTION('',(0.,1.,0.));
#2905=DIRECTION('center_axis',(0.,0.,1.));
#2906=DIRECTION('ref_axis',(1.,0.,0.));
#2907=DIRECTION('center_axis',(0.,0.,1.));
#2908=DIRECTION('ref_axis',(1.,0.,0.));
#2909=DIRECTION('center_axis',(0.,0.,1.));
#2910=DIRECTION('ref_axis',(1.,0.,0.));
#2911=DIRECTION('',(0.,0.,-1.));
#2912=DIRECTION('',(0.,0.,1.));
#2913=DIRECTION('center_axis',(0.,0.,-1.));
#2914=DIRECTION('ref_axis',(1.,0.,0.));
#2915=DIRECTION('center_axis',(1.,0.,0.));
#2916=DIRECTION('ref_axis',(0.,0.,-1.));
#2917=DIRECTION('',(0.,0.,-1.));
#2918=DIRECTION('center_axis',(0.,0.,1.));
#2919=DIRECTION('ref_axis',(1.,0.,0.));
#2920=DIRECTION('center_axis',(0.,0.,1.));
#2921=DIRECTION('ref_axis',(1.,0.,0.));
#2922=DIRECTION('',(0.,0.,1.));
#2923=DIRECTION('center_axis',(1.,0.,0.));
#2924=DIRECTION('ref_axis',(0.,0.,-1.));
#2925=DIRECTION('',(0.,0.,1.));
#2926=DIRECTION('center_axis',(1.,0.,0.));
#2927=DIRECTION('ref_axis',(0.,0.,-1.));
#2928=DIRECTION('',(0.,0.,1.));
#2929=DIRECTION('center_axis',(0.,0.,1.));
#2930=DIRECTION('ref_axis',(1.,0.,0.));
#2931=DIRECTION('center_axis',(0.,0.,1.));
#2932=DIRECTION('ref_axis',(1.,0.,0.));
#2933=DIRECTION('',(0.,0.,1.));
#2934=DIRECTION('center_axis',(1.,0.,0.));
#2935=DIRECTION('ref_axis',(0.,0.,-1.));
#2936=DIRECTION('',(0.,0.,-1.));
#2937=DIRECTION('center_axis',(0.,0.,1.));
#2938=DIRECTION('ref_axis',(1.,0.,0.));
#2939=DIRECTION('',(0.,0.,1.));
#2940=DIRECTION('',(0.,0.,1.));
#2941=DIRECTION('center_axis',(0.,0.,-1.));
#2942=DIRECTION('ref_axis',(1.,0.,0.));
#2943=DIRECTION('center_axis',(0.,0.,-1.));
#2944=DIRECTION('ref_axis',(1.,0.,0.));
#2945=DIRECTION('center_axis',(0.,0.,1.));
#2946=DIRECTION('ref_axis',(1.,0.,0.));
#2947=DIRECTION('center_axis',(0.,0.,1.));
#2948=DIRECTION('ref_axis',(1.,0.,0.));
#2949=DIRECTION('',(0.,0.,1.));
#2950=DIRECTION('center_axis',(1.,0.,0.));
#2951=DIRECTION('ref_axis',(0.,0.,-1.));
#2952=DIRECTION('',(0.,0.,-1.));
#2953=DIRECTION('center_axis',(0.,0.,1.));
#2954=DIRECTION('ref_axis',(1.,0.,0.));
#2955=DIRECTION('',(0.,0.,1.));
#2956=DIRECTION('center_axis',(0.,0.,-1.));
#2957=DIRECTION('ref_axis',(1.,0.,0.));
#2958=DIRECTION('center_axis',(0.,0.,1.));
#2959=DIRECTION('ref_axis',(1.,0.,0.));
#2960=DIRECTION('',(0.,0.,1.));
#2961=DIRECTION('center_axis',(0.,0.,-1.));
#2962=DIRECTION('ref_axis',(1.,0.,0.));
#2963=DIRECTION('center_axis',(1.,0.,0.));
#2964=DIRECTION('ref_axis',(0.,1.,0.));
#2965=DIRECTION('',(0.,0.,1.));
#2966=DIRECTION('',(0.,1.,0.));
#2967=DIRECTION('',(0.,0.,1.));
#2968=DIRECTION('',(0.,-1.,0.));
#2969=DIRECTION('center_axis',(0.,-1.,0.));
#2970=DIRECTION('ref_axis',(1.,0.,0.));
#2971=DIRECTION('',(1.,0.,0.));
#2972=DIRECTION('',(0.,0.,1.));
#2973=DIRECTION('',(1.,0.,0.));
#2974=DIRECTION('center_axis',(0.,0.,1.));
#2975=DIRECTION('ref_axis',(0.,-1.,0.));
#2976=DIRECTION('',(0.,-1.,0.));
#2977=DIRECTION('',(1.,0.,0.));
#2978=DIRECTION('',(0.,-1.,0.));
#2979=DIRECTION('center_axis',(0.,1.,0.));
#2980=DIRECTION('ref_axis',(-1.,0.,0.));
#2981=DIRECTION('',(-1.,0.,0.));
#2982=DIRECTION('',(0.,0.,1.));
#2983=DIRECTION('center_axis',(-1.,0.,0.));
#2984=DIRECTION('ref_axis',(0.,-1.,0.));
#2985=DIRECTION('',(0.,-1.,0.));
#2986=DIRECTION('center_axis',(0.,0.,1.));
#2987=DIRECTION('ref_axis',(1.,0.,0.));
#3528=CARTESIAN_POINT('',(0.,0.,0.));
#3529=CARTESIAN_POINT('Origin',(-1.2,0.,6.));
#3530=CARTESIAN_POINT('',(-1.2,1.26252272915133,4.86156407366234));
#3531=CARTESIAN_POINT('',(-1.2,1.26252272915133,5.));
#3532=CARTESIAN_POINT('',(-1.2,1.26252272915133,4.1));
#3533=CARTESIAN_POINT('',(-1.2,-1.26252272915133,4.86156407366234));
#3534=CARTESIAN_POINT('Origin',(-1.2,0.,6.));
#3535=CARTESIAN_POINT('',(-1.2,-1.26252272915133,5.));
#3536=CARTESIAN_POINT('',(-1.2,-1.26252272915133,4.1));
#3537=CARTESIAN_POINT('',(-1.2,1.25,5.));
#3538=CARTESIAN_POINT('Origin',(-3.6,0.,6.));
#3539=CARTESIAN_POINT('',(-1.82903432003806,1.37477270848678,5.));
#3540=CARTESIAN_POINT('Ctrl Pts',(-1.82903432003806,1.37477270848676,5.00000000000002));
#3541=CARTESIAN_POINT('Ctrl Pts',(-1.82812531946363,1.36291680291864,4.98370082459056));
#3542=CARTESIAN_POINT('Ctrl Pts',(-1.82653488263586,1.35063671201868,4.96743485680573));
#3543=CARTESIAN_POINT('Ctrl Pts',(-1.81822884513887,1.30711001024898,4.91188459887471));
#3544=CARTESIAN_POINT('Ctrl Pts',(-1.80714205446995,1.27468449144834,4.87434693316054));
#3545=CARTESIAN_POINT('Ctrl Pts',(-1.77578652436294,1.21580790152752,4.81103672837552));
#3546=CARTESIAN_POINT('Ctrl Pts',(-1.75030832988751,1.18152448377587,4.77719694611154));
#3547=CARTESIAN_POINT('Ctrl Pts',(-1.69569663875101,1.13196676018157,4.73126383714339));
#3548=CARTESIAN_POINT('Ctrl Pts',(-1.66179162252479,1.10939592163522,4.71172525423958));
#3549=CARTESIAN_POINT('Ctrl Pts',(-1.5846841815694,1.07835439237347,4.6856321341911));
#3550=CARTESIAN_POINT('Ctrl Pts',(-1.54146883053287,1.07,4.67897766862176));
#3551=CARTESIAN_POINT('Ctrl Pts',(-1.45853116946713,1.07,4.67897766862176));
#3552=CARTESIAN_POINT('Ctrl Pts',(-1.4153158184306,1.07835439237347,4.6856321341911));
#3553=CARTESIAN_POINT('Ctrl Pts',(-1.33820837747521,1.10939592163522,4.71172525423958));
#3554=CARTESIAN_POINT('Ctrl Pts',(-1.30430336124899,1.13196676018157,4.73126383714339));
#3555=CARTESIAN_POINT('Ctrl Pts',(-1.24969167011249,1.18152448377587,4.77719694611154));
#3556=CARTESIAN_POINT('Ctrl Pts',(-1.22421347563706,1.21580790152752,4.81103672837552));
#3557=CARTESIAN_POINT('Ctrl Pts',(-1.20564651189243,1.25067127353037,4.84852543524467));
#3558=CARTESIAN_POINT('Ctrl Pts',(-1.20273149014269,1.25656212898995,4.85495378228886));
#3559=CARTESIAN_POINT('Ctrl Pts',(-1.2,1.26252272915133,4.86156407366234));
#3560=CARTESIAN_POINT('',(-2.4511708863178,1.37477270848675,5.));
#3561=CARTESIAN_POINT('',(-3.6,1.37477270848675,5.));
#3562=CARTESIAN_POINT('',(-3.1488291136822,1.37477270848675,5.));
#3563=CARTESIAN_POINT('Ctrl Pts',(-3.1488291136822,1.37477270848675,5.));
#3564=CARTESIAN_POINT('Ctrl Pts',(-3.11342817786855,1.34573205820429,4.96007570655496));
#3565=CARTESIAN_POINT('Ctrl Pts',(-3.06914962012721,1.31716857379013,4.92472362043486));
#3566=CARTESIAN_POINT('Ctrl Pts',(-2.98559269661871,1.28103353525338,4.88222090056834));
#3567=CARTESIAN_POINT('Ctrl Pts',(-2.95013776503027,1.26954894147296,4.86934551918671));
#3568=CARTESIAN_POINT('Ctrl Pts',(-2.87639593827315,1.25402991358996,4.85215722115304));
#3569=CARTESIAN_POINT('Ctrl Pts',(-2.83811186099248,1.25,4.84782813781971));
#3570=CARTESIAN_POINT('Ctrl Pts',(-2.76188813900752,1.25,4.84782813781971));
#3571=CARTESIAN_POINT('Ctrl Pts',(-2.72360406172685,1.25402991358996,4.85215722115304));
#3572=CARTESIAN_POINT('Ctrl Pts',(-2.64986223496973,1.26954894147297,4.86934551918671));
#3573=CARTESIAN_POINT('Ctrl Pts',(-2.61440730338129,1.28103353525338,4.88222090056834));
#3574=CARTESIAN_POINT('Ctrl Pts',(-2.53085037987278,1.31716857379013,4.92472362043486));
#3575=CARTESIAN_POINT('Ctrl Pts',(-2.48657182213145,1.34573205820429,4.96007570655496));
#3576=CARTESIAN_POINT('Ctrl Pts',(-2.4511708863178,1.37477270848675,5.));
#3577=CARTESIAN_POINT('',(-3.5,1.37477270848675,5.));
#3578=CARTESIAN_POINT('',(-3.6,1.37477270848675,5.));
#3579=CARTESIAN_POINT('',(-3.5,-1.37477270848675,5.));
#3580=CARTESIAN_POINT('Origin',(-3.5,0.,6.));
#3581=CARTESIAN_POINT('',(-3.1488291136822,-1.37477270848675,5.));
#3582=CARTESIAN_POINT('',(-3.6,-1.37477270848675,5.));
#3583=CARTESIAN_POINT('',(-2.4511708863178,-1.37477270848675,5.));
#3584=CARTESIAN_POINT('Ctrl Pts',(-2.4511708863178,-1.37477270848675,5.));
#3585=CARTESIAN_POINT('Ctrl Pts',(-2.48657182213145,-1.34573205820429,4.96007570655496));
#3586=CARTESIAN_POINT('Ctrl Pts',(-2.53085037987278,-1.31716857379013,4.92472362043486));
#3587=CARTESIAN_POINT('Ctrl Pts',(-2.61440730338129,-1.28103353525338,4.88222090056834));
#3588=CARTESIAN_POINT('Ctrl Pts',(-2.64986223496973,-1.26954894147297,4.86934551918671));
#3589=CARTESIAN_POINT('Ctrl Pts',(-2.72360406172685,-1.25402991358996,4.85215722115304));
#3590=CARTESIAN_POINT('Ctrl Pts',(-2.76188813900752,-1.25,4.84782813781971));
#3591=CARTESIAN_POINT('Ctrl Pts',(-2.8,-1.25,4.84782813781971));
#3592=CARTESIAN_POINT('Ctrl Pts',(-2.83811186099248,-1.25,4.84782813781971));
#3593=CARTESIAN_POINT('Ctrl Pts',(-2.87639593827315,-1.25402991358996,4.85215722115304));
#3594=CARTESIAN_POINT('Ctrl Pts',(-2.95013776503027,-1.26954894147297,4.86934551918671));
#3595=CARTESIAN_POINT('Ctrl Pts',(-2.98559269661871,-1.28103353525338,4.88222090056834));
#3596=CARTESIAN_POINT('Ctrl Pts',(-3.06914962012721,-1.31716857379013,4.92472362043486));
#3597=CARTESIAN_POINT('Ctrl Pts',(-3.11342817786855,-1.34573205820429,4.96007570655496));
#3598=CARTESIAN_POINT('Ctrl Pts',(-3.1488291136822,-1.37477270848675,5.));
#3599=CARTESIAN_POINT('',(-1.82903432003806,-1.37477270848678,5.));
#3600=CARTESIAN_POINT('',(-3.6,-1.37477270848675,5.));
#3601=CARTESIAN_POINT('Ctrl Pts',(-1.2,-1.26252272915133,4.86156407366234));
#3602=CARTESIAN_POINT('Ctrl Pts',(-1.20273149013951,-1.25656212899688,4.85495378229655));
#3603=CARTESIAN_POINT('Ctrl Pts',(-1.20564651188764,-1.25067127353937,4.84852543525435));
#3604=CARTESIAN_POINT('Ctrl Pts',(-1.22421347563706,-1.21580790152752,4.81103672837552));
#3605=CARTESIAN_POINT('Ctrl Pts',(-1.24969167011249,-1.18152448377587,4.77719694611154));
#3606=CARTESIAN_POINT('Ctrl Pts',(-1.30430336124899,-1.13196676018157,4.73126383714339));
#3607=CARTESIAN_POINT('Ctrl Pts',(-1.33820837747521,-1.10939592163522,4.71172525423958));
#3608=CARTESIAN_POINT('Ctrl Pts',(-1.4153158184306,-1.07835439237347,4.68563213419111));
#3609=CARTESIAN_POINT('Ctrl Pts',(-1.45853116946713,-1.07,4.67897766862176));
#3610=CARTESIAN_POINT('Ctrl Pts',(-1.5,-1.07,4.67897766862176));
#3611=CARTESIAN_POINT('Ctrl Pts',(-1.54146883053287,-1.07,4.67897766862176));
#3612=CARTESIAN_POINT('Ctrl Pts',(-1.5846841815694,-1.07835439237347,4.68563213419111));
#3613=CARTESIAN_POINT('Ctrl Pts',(-1.66179162252479,-1.10939592163522,4.71172525423958));
#3614=CARTESIAN_POINT('Ctrl Pts',(-1.69569663875101,-1.13196676018157,4.73126383714339));
#3615=CARTESIAN_POINT('Ctrl Pts',(-1.75030832988751,-1.18152448377587,4.77719694611154));
#3616=CARTESIAN_POINT('Ctrl Pts',(-1.77578652436294,-1.21580790152752,4.81103672837552));
#3617=CARTESIAN_POINT('Ctrl Pts',(-1.80714205446995,-1.27468449144834,4.87434693316054));
#3618=CARTESIAN_POINT('Ctrl Pts',(-1.81822884513887,-1.30711001024898,4.91188459887471));
#3619=CARTESIAN_POINT('Ctrl Pts',(-1.82653488263586,-1.35063671201868,4.96743485680573));
#3620=CARTESIAN_POINT('Ctrl Pts',(-1.82812531946363,-1.36291680291864,4.98370082459056));
#3621=CARTESIAN_POINT('Ctrl Pts',(-1.82903432003806,-1.37477270848676,5.00000000000002));
#3622=CARTESIAN_POINT('Origin',(-2.8,1.8,0.8));
#3623=CARTESIAN_POINT('',(-2.5,2.26097722286464,4.2));
#3624=CARTESIAN_POINT('',(-2.5,2.26097722286464,0.8));
#3625=CARTESIAN_POINT('',(-2.5,2.26097722286464,0.8));
#3626=CARTESIAN_POINT('',(-2.5,1.33902277713536,4.2));
#3627=CARTESIAN_POINT('Origin',(-2.8,1.8,4.2));
#3628=CARTESIAN_POINT('',(-2.5,1.33902277713536,0.8));
#3629=CARTESIAN_POINT('',(-2.5,1.33902277713536,0.8));
#3630=CARTESIAN_POINT('',(-3.35,1.8,0.8));
#3631=CARTESIAN_POINT('Origin',(-2.8,1.8,0.8));
#3632=CARTESIAN_POINT('',(-3.35,1.8,5.));
#3633=CARTESIAN_POINT('',(-3.35,1.8,0.8));
#3634=CARTESIAN_POINT('Origin',(-2.8,1.8,5.));
#3635=CARTESIAN_POINT('Origin',(-2.8,1.8,5.));
#3636=CARTESIAN_POINT('Origin',(-2.8,1.8,0.8));
#3637=CARTESIAN_POINT('Origin',(-1.5,1.4,4.1));
#3638=CARTESIAN_POINT('',(-1.83,1.4,4.2));
#3639=CARTESIAN_POINT('Origin',(-1.5,1.4,4.2));
#3640=CARTESIAN_POINT('',(-1.83,1.4,5.00000000000002));
#3641=CARTESIAN_POINT('',(-1.83,1.4,4.1));
#3642=CARTESIAN_POINT('Origin',(-1.5,1.4,5.));
#3643=CARTESIAN_POINT('Origin',(-1.5,1.4,5.));
#3644=CARTESIAN_POINT('Origin',(-1.5,-1.4,4.1));
#3645=CARTESIAN_POINT('',(-1.83,-1.4,4.2));
#3646=CARTESIAN_POINT('Origin',(-1.5,-1.4,4.2));
#3647=CARTESIAN_POINT('',(-1.83,-1.4,5.00000000000002));
#3648=CARTESIAN_POINT('',(-1.83,-1.4,4.1));
#3649=CARTESIAN_POINT('Origin',(-1.5,-1.4,5.));
#3650=CARTESIAN_POINT('Origin',(-1.5,-1.4,5.));
#3651=CARTESIAN_POINT('Origin',(2.8,1.8,0.8));
#3652=CARTESIAN_POINT('',(2.5,1.33902277713536,4.2));
#3653=CARTESIAN_POINT('',(2.5,1.33902277713536,0.8));
#3654=CARTESIAN_POINT('',(2.5,1.33902277713536,0.8));
#3655=CARTESIAN_POINT('',(2.25,1.8,4.2));
#3656=CARTESIAN_POINT('Origin',(2.8,1.8,4.2));
#3657=CARTESIAN_POINT('',(2.25,1.8,5.));
#3658=CARTESIAN_POINT('',(2.25,1.8,0.8));
#3659=CARTESIAN_POINT('Origin',(2.8,1.8,5.));
#3660=CARTESIAN_POINT('',(2.5,2.26097722286464,4.2));
#3661=CARTESIAN_POINT('Origin',(2.8,1.8,4.2));
#3662=CARTESIAN_POINT('',(2.5,2.26097722286464,0.8));
#3663=CARTESIAN_POINT('',(2.5,2.26097722286464,0.8));
#3664=CARTESIAN_POINT('Origin',(2.8,1.8,0.8));
#3665=CARTESIAN_POINT('Origin',(2.5,0.,2.85));
#3666=CARTESIAN_POINT('',(2.5,-1.33902277713536,0.8));
#3667=CARTESIAN_POINT('',(2.5,0.,0.8));
#3668=CARTESIAN_POINT('',(2.5,-1.33902277713536,4.2));
#3669=CARTESIAN_POINT('',(2.5,-1.33902277713536,0.8));
#3670=CARTESIAN_POINT('',(2.5,0.,4.2));
#3671=CARTESIAN_POINT('Origin',(0.,0.,0.8));
#3672=CARTESIAN_POINT('',(2.5,2.5,0.8));
#3673=CARTESIAN_POINT('',(2.5,0.,0.8));
#3674=CARTESIAN_POINT('',(-2.5,2.5,0.8));
#3675=CARTESIAN_POINT('',(3.5,2.5,0.8));
#3676=CARTESIAN_POINT('',(-2.5,0.,0.8));
#3677=CARTESIAN_POINT('',(-2.5,-1.33902277713536,0.8));
#3678=CARTESIAN_POINT('',(-2.5,0.,0.8));
#3679=CARTESIAN_POINT('',(-3.35,-1.8,0.8));
#3680=CARTESIAN_POINT('Origin',(-2.8,-1.8,0.8));
#3681=CARTESIAN_POINT('',(-2.5,-2.26097722286464,0.8));
#3682=CARTESIAN_POINT('Origin',(-2.8,-1.8,0.8));
#3683=CARTESIAN_POINT('',(-2.5,-2.5,0.8));
#3684=CARTESIAN_POINT('',(-2.5,0.,0.8));
#3685=CARTESIAN_POINT('',(2.5,-2.5,0.8));
#3686=CARTESIAN_POINT('',(-3.5,-2.5,0.8));
#3687=CARTESIAN_POINT('',(2.5,-2.26097722286464,0.8));
#3688=CARTESIAN_POINT('',(2.5,0.,0.8));
#3689=CARTESIAN_POINT('Origin',(2.8,-1.8,0.8));
#3690=CARTESIAN_POINT('',(2.47,-1.8,0.8));
#3691=CARTESIAN_POINT('Origin',(2.8,-1.8,0.8));
#3692=CARTESIAN_POINT('',(-3.13,-1.8,0.8));
#3693=CARTESIAN_POINT('Origin',(-2.8,-1.8,0.8));
#3694=CARTESIAN_POINT('',(-3.13,1.8,0.8));
#3695=CARTESIAN_POINT('Origin',(-2.8,1.8,0.8));
#3696=CARTESIAN_POINT('',(2.47,1.8,0.8));
#3697=CARTESIAN_POINT('Origin',(2.8,1.8,0.8));
#3698=CARTESIAN_POINT('Origin',(2.8,1.8,-0.1));
#3699=CARTESIAN_POINT('',(2.47,1.8,0.));
#3700=CARTESIAN_POINT('Origin',(2.8,1.8,0.));
#3701=CARTESIAN_POINT('',(2.47,1.8,-0.1));
#3702=CARTESIAN_POINT('Origin',(0.,0.,4.2));
#3703=CARTESIAN_POINT('',(2.25,-1.8,4.2));
#3704=CARTESIAN_POINT('Origin',(2.8,-1.8,4.2));
#3705=CARTESIAN_POINT('',(2.5,-2.26097722286464,4.2));
#3706=CARTESIAN_POINT('Origin',(2.8,-1.8,4.2));
#3707=CARTESIAN_POINT('',(2.5,-2.5,4.2));
#3708=CARTESIAN_POINT('',(2.5,0.,4.2));
#3709=CARTESIAN_POINT('',(-2.5,-2.5,4.2));
#3710=CARTESIAN_POINT('',(-3.5,-2.5,4.2));
#3711=CARTESIAN_POINT('',(-2.5,-2.26097722286464,4.2));
#3712=CARTESIAN_POINT('',(-2.5,0.,4.2));
#3713=CARTESIAN_POINT('',(-2.5,-1.33902277713536,4.2));
#3714=CARTESIAN_POINT('Origin',(-2.8,-1.8,4.2));
#3715=CARTESIAN_POINT('',(-2.5,0.,4.2));
#3716=CARTESIAN_POINT('',(-2.5,2.5,4.2));
#3717=CARTESIAN_POINT('',(-2.5,0.,4.2));
#3718=CARTESIAN_POINT('',(2.5,2.5,4.2));
#3719=CARTESIAN_POINT('',(3.5,2.5,4.2));
#3720=CARTESIAN_POINT('',(2.5,0.,4.2));
#3721=CARTESIAN_POINT('',(1.17,-1.4,4.2));
#3722=CARTESIAN_POINT('Origin',(1.5,-1.4,4.2));
#3723=CARTESIAN_POINT('',(1.17,1.4,4.2));
#3724=CARTESIAN_POINT('Origin',(1.5,1.4,4.2));
#3725=CARTESIAN_POINT('Origin',(2.8,-1.8,0.8));
#3726=CARTESIAN_POINT('',(2.5,-2.26097722286464,0.8));
#3727=CARTESIAN_POINT('',(2.25,-1.8,5.));
#3728=CARTESIAN_POINT('',(2.25,-1.8,0.8));
#3729=CARTESIAN_POINT('Origin',(2.8,-1.8,5.));
#3730=CARTESIAN_POINT('Origin',(2.5,0.,2.85));
#3731=CARTESIAN_POINT('',(2.5,-2.5,5.));
#3732=CARTESIAN_POINT('Origin',(2.8,-1.8,-0.1));
#3733=CARTESIAN_POINT('',(2.47,-1.8,0.));
#3734=CARTESIAN_POINT('Origin',(2.8,-1.8,0.));
#3735=CARTESIAN_POINT('',(2.47,-1.8,-0.1));
#3736=CARTESIAN_POINT('Origin',(2.5,0.,2.85));
#3737=CARTESIAN_POINT('',(2.5,2.5,0.7));
#3738=CARTESIAN_POINT('Origin',(-2.5,0.,2.85));
#3739=CARTESIAN_POINT('',(-2.5,2.5,0.7));
#3740=CARTESIAN_POINT('Origin',(-2.8,1.8,-0.1));
#3741=CARTESIAN_POINT('',(-3.13,1.8,0.));
#3742=CARTESIAN_POINT('Origin',(-2.8,1.8,0.));
#3743=CARTESIAN_POINT('',(-3.13,1.8,-0.1));
#3744=CARTESIAN_POINT('Origin',(-2.5,0.,2.85));
#3745=CARTESIAN_POINT('',(-2.5,-1.33902277713536,0.8));
#3746=CARTESIAN_POINT('Origin',(-2.8,-1.8,0.8));
#3747=CARTESIAN_POINT('',(-2.5,-2.26097722286464,0.8));
#3748=CARTESIAN_POINT('',(-3.35,-1.8,5.));
#3749=CARTESIAN_POINT('',(-3.35,-1.8,0.8));
#3750=CARTESIAN_POINT('Origin',(-2.8,-1.8,5.));
#3751=CARTESIAN_POINT('Origin',(-2.8,-1.8,5.));
#3752=CARTESIAN_POINT('Origin',(-2.8,-1.8,-0.1));
#3753=CARTESIAN_POINT('',(-3.13,-1.8,0.));
#3754=CARTESIAN_POINT('Origin',(-2.8,-1.8,0.));
#3755=CARTESIAN_POINT('',(-3.13,-1.8,-0.1));
#3756=CARTESIAN_POINT('Origin',(-2.5,0.,2.85));
#3757=CARTESIAN_POINT('',(-2.5,-2.5,5.));
#3758=CARTESIAN_POINT('Origin',(1.5,1.4,4.1));
#3759=CARTESIAN_POINT('',(1.17,1.4,5.));
#3760=CARTESIAN_POINT('',(1.17,1.4,4.1));
#3761=CARTESIAN_POINT('Origin',(1.5,1.4,5.));
#3762=CARTESIAN_POINT('Origin',(1.5,-1.4,4.1));
#3763=CARTESIAN_POINT('',(1.17,-1.4,5.));
#3764=CARTESIAN_POINT('',(1.17,-1.4,4.1));
#3765=CARTESIAN_POINT('Origin',(1.5,-1.4,5.));
#3766=CARTESIAN_POINT('Origin',(3.5,-2.5,0.));
#3767=CARTESIAN_POINT('',(3.5,-2.5,0.));
#3768=CARTESIAN_POINT('',(3.5,-2.5,5.));
#3769=CARTESIAN_POINT('',(3.5,-2.5,0.));
#3770=CARTESIAN_POINT('',(3.5,2.5,0.));
#3771=CARTESIAN_POINT('',(3.5,-2.5,0.));
#3772=CARTESIAN_POINT('',(3.5,2.5,5.));
#3773=CARTESIAN_POINT('',(3.5,2.5,0.));
#3774=CARTESIAN_POINT('',(3.5,2.5,5.));
#3775=CARTESIAN_POINT('Origin',(-3.5,-2.5,0.));
#3776=CARTESIAN_POINT('',(-3.5,-2.5,5.));
#3777=CARTESIAN_POINT('',(-3.5,-2.5,5.));
#3778=CARTESIAN_POINT('',(-3.5,-2.5,0.));
#3779=CARTESIAN_POINT('',(-3.5,-2.5,0.));
#3780=CARTESIAN_POINT('',(-3.5,-2.5,0.));
#3781=CARTESIAN_POINT('Origin',(2.5,2.5,5.));
#3782=CARTESIAN_POINT('',(-3.5,2.5,5.));
#3783=CARTESIAN_POINT('',(-3.5,2.5,5.));
#3784=CARTESIAN_POINT('',(2.5,2.5,5.));
#3785=CARTESIAN_POINT('',(-3.5,2.5,5.));
#3786=CARTESIAN_POINT('Origin',(3.5,2.5,0.));
#3787=CARTESIAN_POINT('',(-3.5,2.5,0.));
#3788=CARTESIAN_POINT('',(3.5,2.5,0.));
#3789=CARTESIAN_POINT('',(-3.5,2.5,0.));
#3790=CARTESIAN_POINT('Origin',(-3.5,2.5,0.));
#3791=CARTESIAN_POINT('',(-3.5,2.5,0.));
#3792=CARTESIAN_POINT('Origin',(0.,0.,0.));
#4026=UNCERTAINTY_MEASURE_WITH_UNIT(LENGTH_MEASURE(0.001),#4044,
'DISTANCE_ACCURACY_VALUE',
'Maximum model space distance between geometric entities at asserted c
onnectivities');
#4032=UNCERTAINTY_MEASURE_WITH_UNIT(LENGTH_MEASURE(0.001),#4044,
'DISTANCE_ACCURACY_VALUE',
'Maximum model space distance between geometric entities at asserted c
onnectivities');
#4037=(
GEOMETRIC_REPRESENTATION_CONTEXT(3)
GLOBAL_UNCERTAINTY_ASSIGNED_CONTEXT((#4026))
GLOBAL_UNIT_ASSIGNED_CONTEXT((#4044,#4046,#4047))
REPRESENTATION_CONTEXT('','3D')
);
#4043=(
GEOMETRIC_REPRESENTATION_CONTEXT(3)
GLOBAL_UNCERTAINTY_ASSIGNED_CONTEXT((#4032))
GLOBAL_UNIT_ASSIGNED_CONTEXT((#4044,#4046,#4047))
REPRESENTATION_CONTEXT('','3D')
);
#4044=(
LENGTH_UNIT()
NAMED_UNIT(*)
SI_UNIT(.CENTI.,.METRE.)
);
#4046=(
NAMED_UNIT(*)
PLANE_ANGLE_UNIT()
SI_UNIT($,.RADIAN.)
);
#4047=(
NAMED_UNIT(*)
SI_UNIT($,.STERADIAN.)
SOLID_ANGLE_UNIT()
);
#4052=SHAPE_DEFINITION_REPRESENTATION(#4062,#4085);
#4062=PRODUCT_DEFINITION_SHAPE('',$,#4096);
#4085=SHAPE_REPRESENTATION('',(#2400),#4037);
#4091=PRODUCT_DEFINITION_CONTEXT('part definition',#4123,'design');
#4096=PRODUCT_DEFINITION('Valve mounting saddle',
'Valve mounting saddle',#4106,#4091);
#4106=PRODUCT_DEFINITION_FORMATION('',$,#4129);
#4123=APPLICATION_CONTEXT(
'Core Data for Automotive Mechanical Design Process');
#4124=PRODUCT_CONTEXT('part definition',#4123,'mechanical');
#4129=PRODUCT('Valve mounting saddle','Valve mounting saddle',
'Valve mounting saddle',(#4124));
#4205=COLOUR_RGB('Off White',0.89,0.88,0.83);
#4206=FILL_AREA_STYLE_COLOUR('',#4205);
#4207=FILL_AREA_STYLE('',(#4206));
#4208=SURFACE_STYLE_FILL_AREA(#4207);
#4209=SURFACE_SIDE_STYLE('',(#4208));
#4210=SURFACE_STYLE_USAGE(.BOTH.,#4209);
#4211=PRESENTATION_STYLE_ASSIGNMENT((#4210));
ENDSEC;
END-ISO-10303-21;
